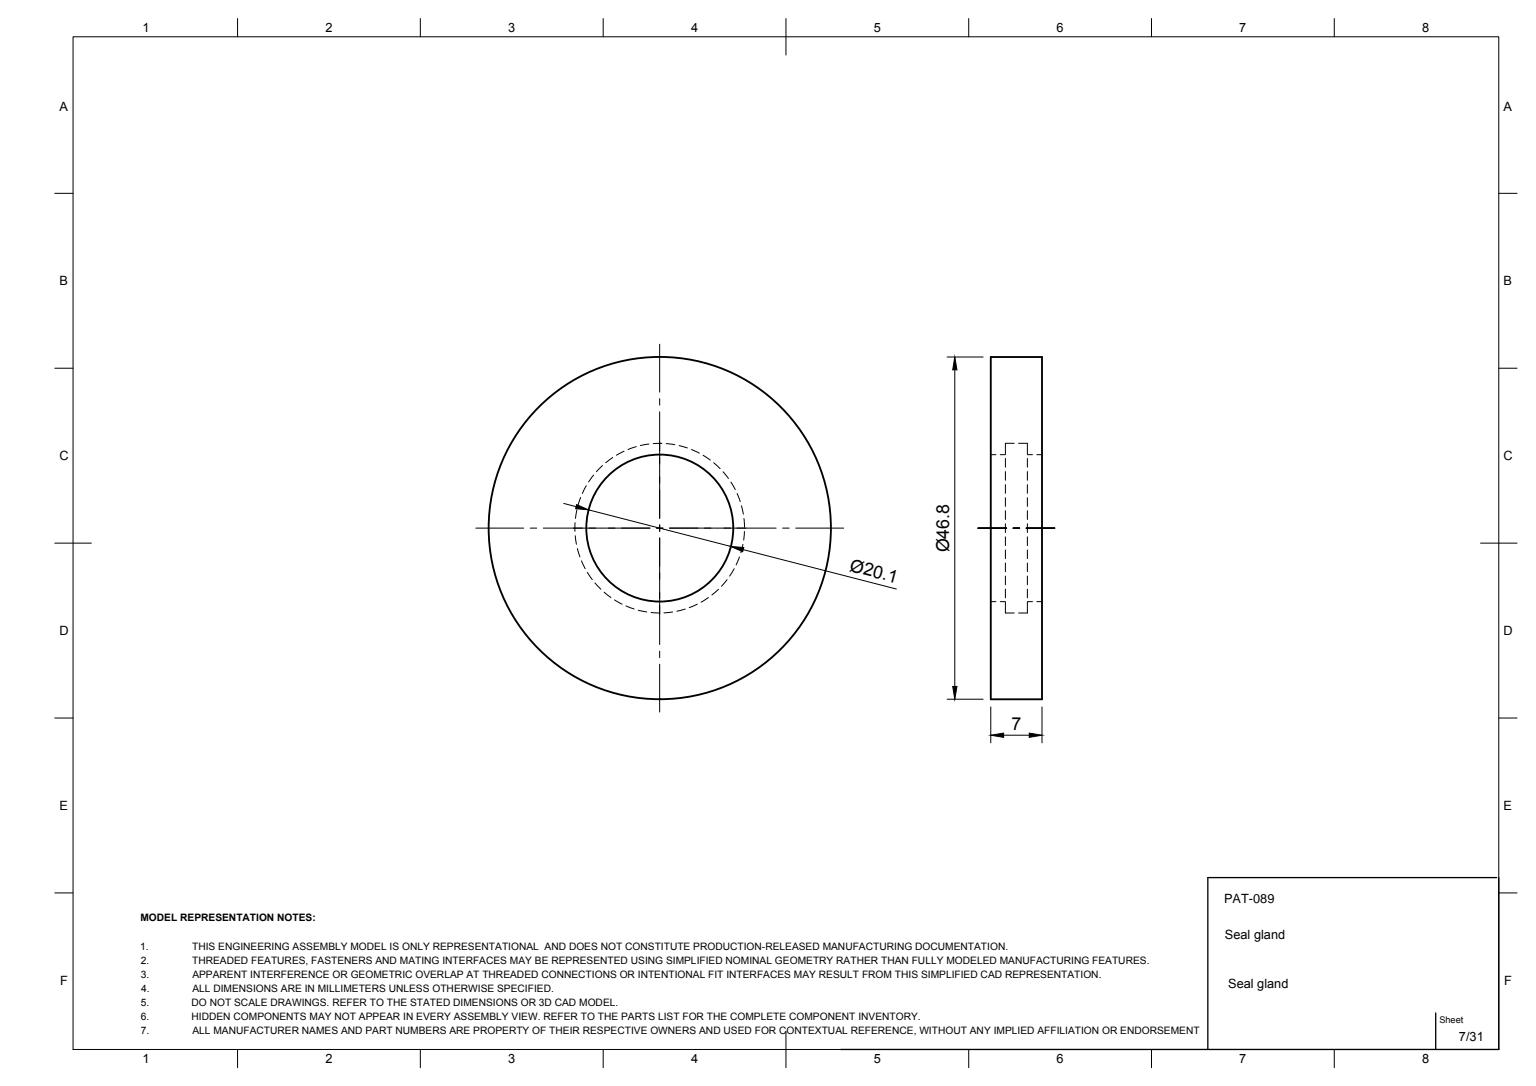
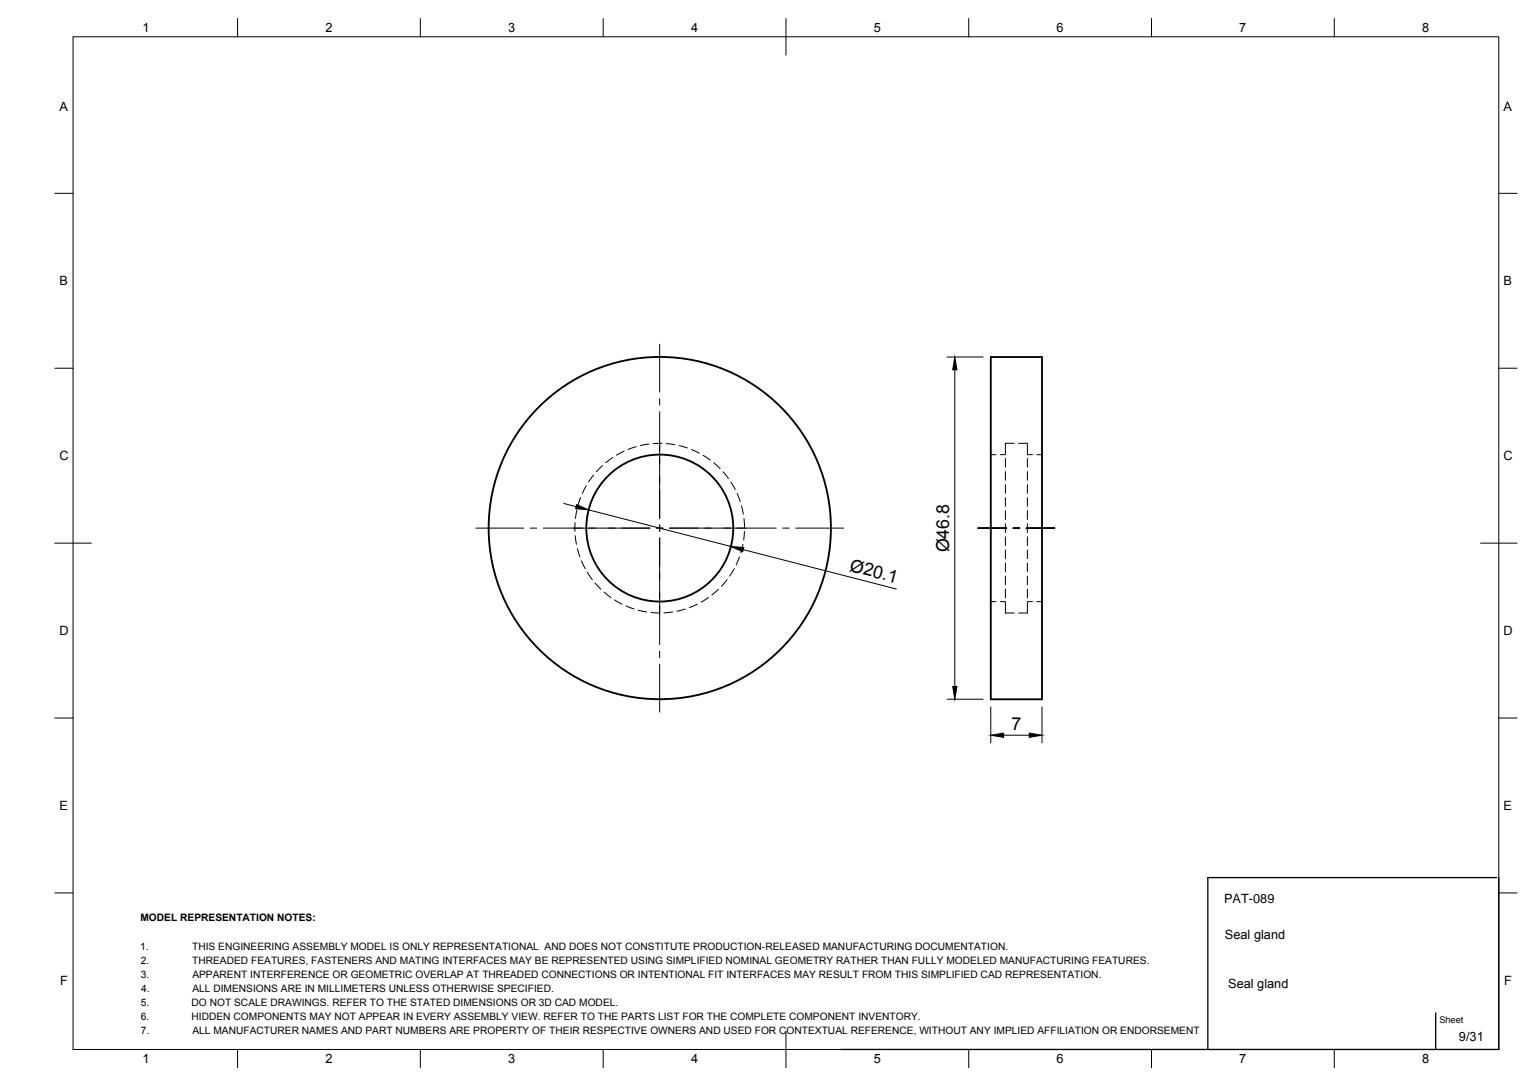
ISO-10303-21;
HEADER;
/* Generated by software containing ST-Developer
 * from STEP Tools, Inc. (www.steptools.com) 
 */

FILE_DESCRIPTION(
/* description */ ('Rotary union on bearing shaft'),
/* implementation_level */ '2;1');

FILE_NAME(
/* name */ 'Seal gland.step',
/* time_stamp */ '2026-10-28T03:24:01-07:00',
/* author */ (''),
/* organization */ (''),
/* preprocessor_version */ 'ST-DEVELOPER v20.2',
/* originating_system */ 'Autodesk Translation Framework v15.17.0.0',
/* authorisation */ '');

FILE_SCHEMA (('AUTOMOTIVE_DESIGN { 1 0 10303 214 3 1 1 }'));
ENDSEC;

DATA;
#10=MECHANICAL_DESIGN_GEOMETRIC_PRESENTATION_REPRESENTATION('',(#315),#9448);
#261=SHAPE_REPRESENTATION_RELATIONSHIP('SRR','None',#9561,#288);
#288=ADVANCED_BREP_SHAPE_REPRESENTATION('',(#350),#9421);
#315=STYLED_ITEM('',(#9785),#350);
#350=MANIFOLD_SOLID_BREP('Body1',#4870);
#410=FACE_BOUND('',#1040,.T.);
#411=FACE_BOUND('',#1042,.T.);
#412=FACE_BOUND('',#1047,.T.);
#413=FACE_BOUND('',#1049,.T.);
#521=PLANE('',#5309);
#522=PLANE('',#5311);
#523=PLANE('',#5320);
#524=PLANE('',#5321);
#709=FACE_OUTER_BOUND('',#1038,.T.);
#710=FACE_OUTER_BOUND('',#1039,.T.);
#711=FACE_OUTER_BOUND('',#1041,.T.);
#712=FACE_OUTER_BOUND('',#1043,.T.);
#713=FACE_OUTER_BOUND('',#1044,.T.);
#714=FACE_OUTER_BOUND('',#1045,.T.);
#715=FACE_OUTER_BOUND('',#1046,.T.);
#716=FACE_OUTER_BOUND('',#1048,.T.);
#1038=EDGE_LOOP('',(#3497,#3498,#3499,#3500));
#1039=EDGE_LOOP('',(#3501));
#1040=EDGE_LOOP('',(#3502));
#1041=EDGE_LOOP('',(#3503));
#1042=EDGE_LOOP('',(#3504));
#1043=EDGE_LOOP('',(#3505,#3506,#3507,#3508));
#1044=EDGE_LOOP('',(#3509,#3510,#3511,#3512));
#1045=EDGE_LOOP('',(#3513,#3514,#3515,#3516));
#1046=EDGE_LOOP('',(#3517));
#1047=EDGE_LOOP('',(#3518));
#1048=EDGE_LOOP('',(#3519));
#1049=EDGE_LOOP('',(#3520));
#1428=LINE('',#7717,#1748);
#1429=LINE('',#7727,#1749);
#1430=LINE('',#7732,#1750);
#1431=LINE('',#7737,#1751);
#1748=VECTOR('',#6103,1.16);
#1749=VECTOR('',#6116,1.005);
#1750=VECTOR('',#6123,1.005);
#1751=VECTOR('',#6128,2.34);
#2045=CIRCLE('',#5307,1.16);
#2046=CIRCLE('',#5308,1.16);
#2047=CIRCLE('',#5310,1.005);
#2048=CIRCLE('',#5312,1.005);
#2049=CIRCLE('',#5314,1.005);
#2050=CIRCLE('',#5316,1.005);
#2051=CIRCLE('',#5318,2.34);
#2052=CIRCLE('',#5319,2.34);
#2329=VERTEX_POINT('',#7714);
#2330=VERTEX_POINT('',#7716);
#2331=VERTEX_POINT('',#7720);
#2332=VERTEX_POINT('',#7723);
#2333=VERTEX_POINT('',#7726);
#2334=VERTEX_POINT('',#7730);
#2335=VERTEX_POINT('',#7734);
#2336=VERTEX_POINT('',#7736);
#2776=EDGE_CURVE('',#2329,#2329,#2045,.T.);
#2777=EDGE_CURVE('',#2329,#2330,#1428,.T.);
#2778=EDGE_CURVE('',#2330,#2330,#2046,.T.);
#2779=EDGE_CURVE('',#2331,#2331,#2047,.T.);
#2780=EDGE_CURVE('',#2332,#2332,#2048,.T.);
#2781=EDGE_CURVE('',#2332,#2333,#1429,.T.);
#2782=EDGE_CURVE('',#2333,#2333,#2049,.T.);
#2783=EDGE_CURVE('',#2334,#2334,#2050,.T.);
#2784=EDGE_CURVE('',#2334,#2331,#1430,.T.);
#2785=EDGE_CURVE('',#2335,#2335,#2051,.T.);
#2786=EDGE_CURVE('',#2335,#2336,#1431,.T.);
#2787=EDGE_CURVE('',#2336,#2336,#2052,.T.);
#3497=ORIENTED_EDGE('',*,*,#2776,.F.);
#3498=ORIENTED_EDGE('',*,*,#2777,.T.);
#3499=ORIENTED_EDGE('',*,*,#2778,.T.);
#3500=ORIENTED_EDGE('',*,*,#2777,.F.);
#3501=ORIENTED_EDGE('',*,*,#2778,.F.);
#3502=ORIENTED_EDGE('',*,*,#2779,.F.);
#3503=ORIENTED_EDGE('',*,*,#2776,.T.);
#3504=ORIENTED_EDGE('',*,*,#2780,.F.);
#3505=ORIENTED_EDGE('',*,*,#2780,.T.);
#3506=ORIENTED_EDGE('',*,*,#2781,.T.);
#3507=ORIENTED_EDGE('',*,*,#2782,.T.);
#3508=ORIENTED_EDGE('',*,*,#2781,.F.);
#3509=ORIENTED_EDGE('',*,*,#2783,.F.);
#3510=ORIENTED_EDGE('',*,*,#2784,.T.);
#3511=ORIENTED_EDGE('',*,*,#2779,.T.);
#3512=ORIENTED_EDGE('',*,*,#2784,.F.);
#3513=ORIENTED_EDGE('',*,*,#2785,.F.);
#3514=ORIENTED_EDGE('',*,*,#2786,.T.);
#3515=ORIENTED_EDGE('',*,*,#2787,.T.);
#3516=ORIENTED_EDGE('',*,*,#2786,.F.);
#3517=ORIENTED_EDGE('',*,*,#2785,.T.);
#3518=ORIENTED_EDGE('',*,*,#2783,.T.);
#3519=ORIENTED_EDGE('',*,*,#2787,.F.);
#3520=ORIENTED_EDGE('',*,*,#2782,.F.);
#4498=CYLINDRICAL_SURFACE('',#5306,1.16);
#4499=CYLINDRICAL_SURFACE('',#5313,1.005);
#4500=CYLINDRICAL_SURFACE('',#5315,1.005);
#4501=CYLINDRICAL_SURFACE('',#5317,2.34);
#4622=ADVANCED_FACE('',(#709),#4498,.F.);
#4623=ADVANCED_FACE('',(#710,#410),#521,.F.);
#4624=ADVANCED_FACE('',(#711,#411),#522,.T.);
#4625=ADVANCED_FACE('',(#712),#4499,.F.);
#4626=ADVANCED_FACE('',(#713),#4500,.F.);
#4627=ADVANCED_FACE('',(#714),#4501,.T.);
#4628=ADVANCED_FACE('',(#715,#412),#523,.T.);
#4629=ADVANCED_FACE('',(#716,#413),#524,.F.);
#4870=CLOSED_SHELL('',(#4622,#4623,#4624,#4625,#4626,#4627,#4628,#4629));
#5305=AXIS2_PLACEMENT_3D('',#7712,#6097,#6098);
#5306=AXIS2_PLACEMENT_3D('',#7713,#6099,#6100);
#5307=AXIS2_PLACEMENT_3D('',#7715,#6101,#6102);
#5308=AXIS2_PLACEMENT_3D('',#7718,#6104,#6105);
#5309=AXIS2_PLACEMENT_3D('',#7719,#6106,#6107);
#5310=AXIS2_PLACEMENT_3D('',#7721,#6108,#6109);
#5311=AXIS2_PLACEMENT_3D('',#7722,#6110,#6111);
#5312=AXIS2_PLACEMENT_3D('',#7724,#6112,#6113);
#5313=AXIS2_PLACEMENT_3D('',#7725,#6114,#6115);
#5314=AXIS2_PLACEMENT_3D('',#7728,#6117,#6118);
#5315=AXIS2_PLACEMENT_3D('',#7729,#6119,#6120);
#5316=AXIS2_PLACEMENT_3D('',#7731,#6121,#6122);
#5317=AXIS2_PLACEMENT_3D('',#7733,#6124,#6125);
#5318=AXIS2_PLACEMENT_3D('',#7735,#6126,#6127);
#5319=AXIS2_PLACEMENT_3D('',#7738,#6129,#6130);
#5320=AXIS2_PLACEMENT_3D('',#7739,#6131,#6132);
#5321=AXIS2_PLACEMENT_3D('',#7740,#6133,#6134);
#6097=DIRECTION('axis',(0.,0.,1.));
#6098=DIRECTION('refdir',(1.,0.,0.));
#6099=DIRECTION('center_axis',(0.,1.,0.));
#6100=DIRECTION('ref_axis',(1.,0.,0.));
#6101=DIRECTION('center_axis',(0.,1.,0.));
#6102=DIRECTION('ref_axis',(1.,0.,0.));
#6103=DIRECTION('',(0.,1.,0.));
#6104=DIRECTION('center_axis',(0.,1.,0.));
#6105=DIRECTION('ref_axis',(1.,0.,0.));
#6106=DIRECTION('center_axis',(0.,1.,0.));
#6107=DIRECTION('ref_axis',(1.,0.,0.));
#6108=DIRECTION('center_axis',(0.,-1.,0.));
#6109=DIRECTION('ref_axis',(1.,0.,0.));
#6110=DIRECTION('center_axis',(0.,1.,0.));
#6111=DIRECTION('ref_axis',(1.,0.,0.));
#6112=DIRECTION('center_axis',(0.,1.,0.));
#6113=DIRECTION('ref_axis',(1.,0.,0.));
#6114=DIRECTION('center_axis',(0.,1.,0.));
#6115=DIRECTION('ref_axis',(1.,0.,0.));
#6116=DIRECTION('',(0.,-1.,0.));
#6117=DIRECTION('center_axis',(0.,-1.,0.));
#6118=DIRECTION('ref_axis',(1.,0.,0.));
#6119=DIRECTION('center_axis',(0.,1.,0.));
#6120=DIRECTION('ref_axis',(1.,0.,0.));
#6121=DIRECTION('center_axis',(0.,-1.,0.));
#6122=DIRECTION('ref_axis',(1.,0.,0.));
#6123=DIRECTION('',(0.,-1.,0.));
#6124=DIRECTION('center_axis',(0.,1.,0.));
#6125=DIRECTION('ref_axis',(1.,0.,0.));
#6126=DIRECTION('center_axis',(0.,1.,0.));
#6127=DIRECTION('ref_axis',(1.,0.,0.));
#6128=DIRECTION('',(0.,-1.,0.));
#6129=DIRECTION('center_axis',(0.,1.,0.));
#6130=DIRECTION('ref_axis',(1.,0.,0.));
#6131=DIRECTION('center_axis',(0.,1.,0.));
#6132=DIRECTION('ref_axis',(1.,0.,0.));
#6133=DIRECTION('center_axis',(0.,1.,0.));
#6134=DIRECTION('ref_axis',(1.,0.,0.));
#7712=CARTESIAN_POINT('',(0.,0.,0.));
#7713=CARTESIAN_POINT('Origin',(0.,1.9,4.5));
#7714=CARTESIAN_POINT('',(-1.16,1.9,4.5));
#7715=CARTESIAN_POINT('Origin',(0.,1.9,4.5));
#7716=CARTESIAN_POINT('',(-1.16,2.2,4.5));
#7717=CARTESIAN_POINT('',(-1.16,1.9,4.5));
#7718=CARTESIAN_POINT('Origin',(0.,2.2,4.5));
#7719=CARTESIAN_POINT('Origin',(0.,2.2,4.5));
#7720=CARTESIAN_POINT('',(-1.005,2.2,4.5));
#7721=CARTESIAN_POINT('Origin',(0.,2.2,4.5));
#7722=CARTESIAN_POINT('Origin',(0.,1.9,4.5));
#7723=CARTESIAN_POINT('',(-1.005,1.9,4.5));
#7724=CARTESIAN_POINT('Origin',(0.,1.9,4.5));
#7725=CARTESIAN_POINT('Origin',(0.,1.7,4.5));
#7726=CARTESIAN_POINT('',(-1.005,1.7,4.5));
#7727=CARTESIAN_POINT('',(-1.005,1.7,4.5));
#7728=CARTESIAN_POINT('Origin',(0.,1.7,4.5));
#7729=CARTESIAN_POINT('Origin',(0.,1.7,4.5));
#7730=CARTESIAN_POINT('',(-1.005,2.4,4.5));
#7731=CARTESIAN_POINT('Origin',(0.,2.4,4.5));
#7732=CARTESIAN_POINT('',(-1.005,1.7,4.5));
#7733=CARTESIAN_POINT('Origin',(0.,1.7,4.5));
#7734=CARTESIAN_POINT('',(-2.34,2.4,4.5));
#7735=CARTESIAN_POINT('Origin',(0.,2.4,4.5));
#7736=CARTESIAN_POINT('',(-2.34,1.7,4.5));
#7737=CARTESIAN_POINT('',(-2.34,1.7,4.5));
#7738=CARTESIAN_POINT('Origin',(0.,1.7,4.5));
#7739=CARTESIAN_POINT('Origin',(0.,2.4,4.5));
#7740=CARTESIAN_POINT('Origin',(0.,1.7,4.5));
#9389=UNCERTAINTY_MEASURE_WITH_UNIT(LENGTH_MEASURE(0.001),#9449,
'DISTANCE_ACCURACY_VALUE',
'Maximum model space distance between geometric entities at asserted c
onnectivities');
#9416=UNCERTAINTY_MEASURE_WITH_UNIT(LENGTH_MEASURE(0.001),#9449,
'DISTANCE_ACCURACY_VALUE',
'Maximum model space distance between geometric entities at asserted c
onnectivities');
#9421=(
GEOMETRIC_REPRESENTATION_CONTEXT(3)
GLOBAL_UNCERTAINTY_ASSIGNED_CONTEXT((#9389))
GLOBAL_UNIT_ASSIGNED_CONTEXT((#9449,#9451,#9452))
REPRESENTATION_CONTEXT('','3D')
);
#9448=(
GEOMETRIC_REPRESENTATION_CONTEXT(3)
GLOBAL_UNCERTAINTY_ASSIGNED_CONTEXT((#9416))
GLOBAL_UNIT_ASSIGNED_CONTEXT((#9449,#9451,#9452))
REPRESENTATION_CONTEXT('','3D')
);
#9449=(
LENGTH_UNIT()
NAMED_UNIT(*)
SI_UNIT(.CENTI.,.METRE.)
);
#9451=(
NAMED_UNIT(*)
PLANE_ANGLE_UNIT()
SI_UNIT($,.RADIAN.)
);
#9452=(
NAMED_UNIT(*)
SI_UNIT($,.STERADIAN.)
SOLID_ANGLE_UNIT()
);
#9457=SHAPE_DEFINITION_REPRESENTATION(#9488,#9561);
#9488=PRODUCT_DEFINITION_SHAPE('',$,#9593);
#9561=SHAPE_REPRESENTATION('',(#5305),#9421);
#9588=PRODUCT_DEFINITION_CONTEXT('part definition',#9683,'design');
#9593=PRODUCT_DEFINITION('Seal gland','Seal gland',#9624,#9588);
#9624=PRODUCT_DEFINITION_FORMATION('',$,#9689);
#9683=APPLICATION_CONTEXT(
'Core Data for Automotive Mechanical Design Process');
#9684=PRODUCT_CONTEXT('part definition',#9683,'mechanical');
#9689=PRODUCT('Seal gland','Seal gland','Seal gland',(#9684));
#9779=COLOUR_RGB('Black',0.12,0.14,0.17);
#9780=FILL_AREA_STYLE_COLOUR('',#9779);
#9781=FILL_AREA_STYLE('',(#9780));
#9782=SURFACE_STYLE_FILL_AREA(#9781);
#9783=SURFACE_SIDE_STYLE('',(#9782));
#9784=SURFACE_STYLE_USAGE(.BOTH.,#9783);
#9785=PRESENTATION_STYLE_ASSIGNMENT((#9784));
ENDSEC;
END-ISO-10303-21;
